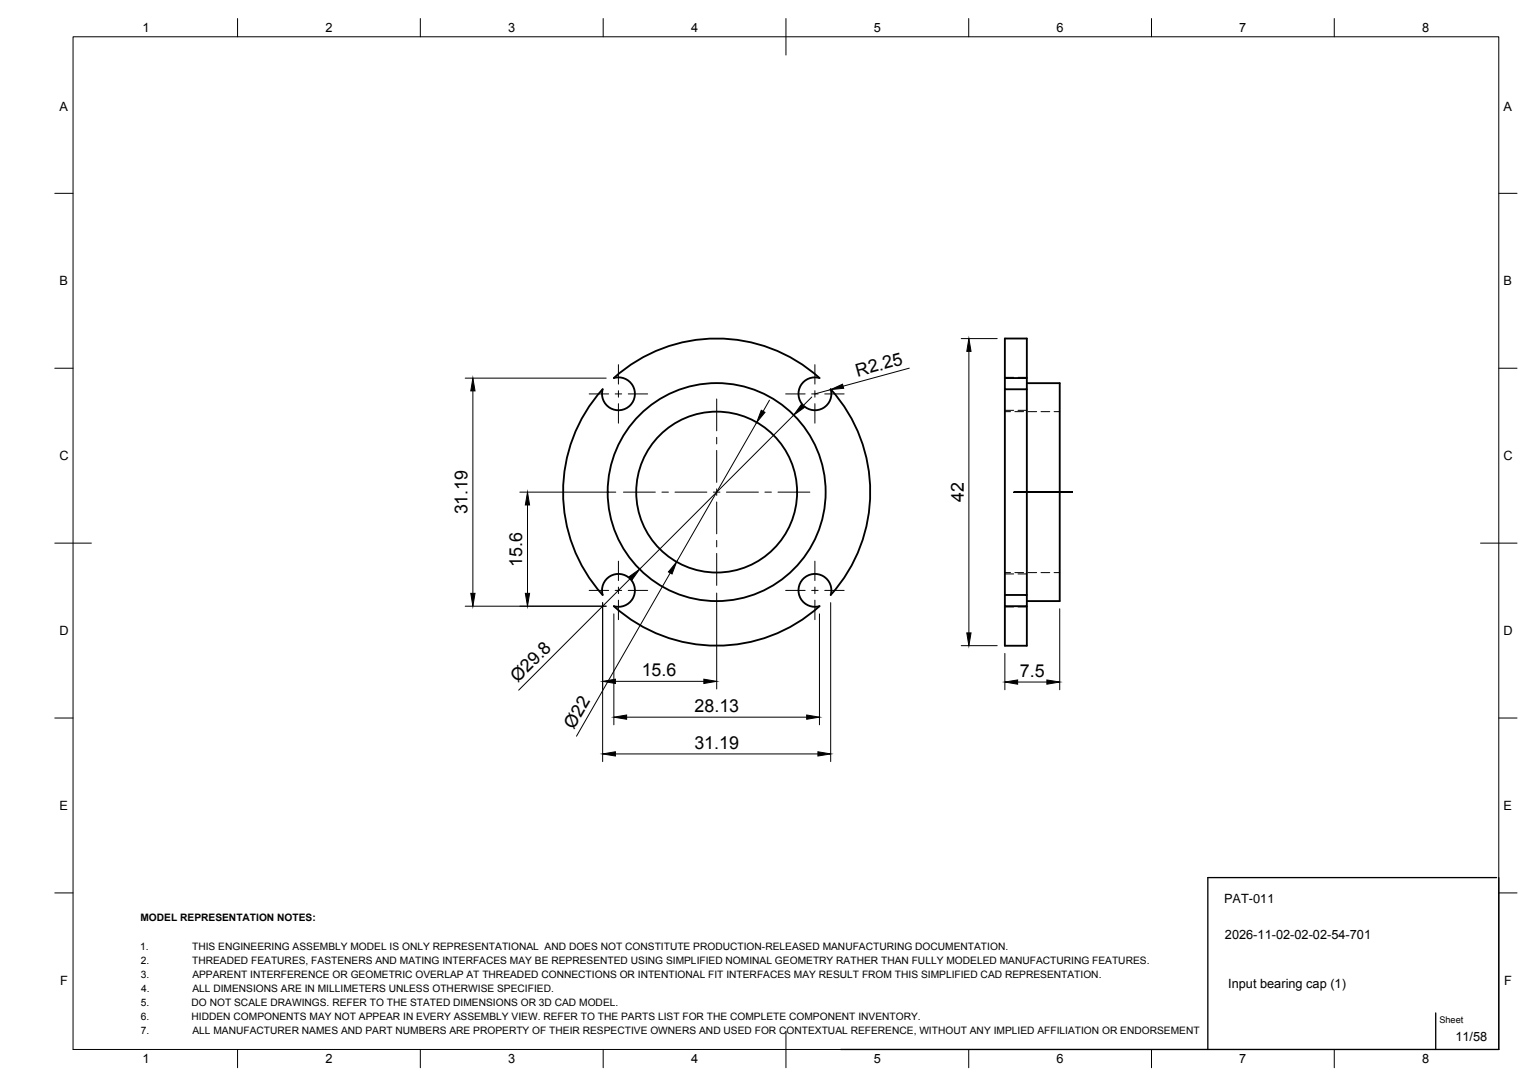
ISO-10303-21;
HEADER;
/* Generated by software containing ST-Developer
 * from STEP Tools, Inc. (www.steptools.com) 
 */

FILE_DESCRIPTION(
/* description */ ('Belt tension measurement rig'),
/* implementation_level */ '2;1');

FILE_NAME(
/* name */ 'Input bearing cap (1).step',
/* time_stamp */ '2026-10-28T03:24:44-07:00',
/* author */ (''),
/* organization */ (''),
/* preprocessor_version */ 'ST-DEVELOPER v20.2',
/* originating_system */ 'Autodesk Translation Framework v15.17.0.0',
/* authorisation */ '');

FILE_SCHEMA (('AUTOMOTIVE_DESIGN { 1 0 10303 214 3 1 1 }'));
ENDSEC;

DATA;
#10=MECHANICAL_DESIGN_GEOMETRIC_PRESENTATION_REPRESENTATION('',(#698),#23587);
#588=SHAPE_REPRESENTATION_RELATIONSHIP('SRR','None',#23833,#643);
#643=ADVANCED_BREP_SHAPE_REPRESENTATION('',(#768),#23531);
#698=STYLED_ITEM('',(#24211),#768);
#768=MANIFOLD_SOLID_BREP('Body1',#12203);
#866=FACE_BOUND('',#2180,.T.);
#867=FACE_BOUND('',#2187,.T.);
#868=FACE_BOUND('',#2190,.T.);
#1084=PLANE('',#13049);
#1085=PLANE('',#13065);
#1086=PLANE('',#13069);
#1434=FACE_OUTER_BOUND('',#2175,.T.);
#1435=FACE_OUTER_BOUND('',#2176,.T.);
#1436=FACE_OUTER_BOUND('',#2177,.T.);
#1437=FACE_OUTER_BOUND('',#2178,.T.);
#1438=FACE_OUTER_BOUND('',#2179,.T.);
#1439=FACE_OUTER_BOUND('',#2181,.T.);
#1440=FACE_OUTER_BOUND('',#2182,.T.);
#1441=FACE_OUTER_BOUND('',#2183,.T.);
#1442=FACE_OUTER_BOUND('',#2184,.T.);
#1443=FACE_OUTER_BOUND('',#2185,.T.);
#1444=FACE_OUTER_BOUND('',#2186,.T.);
#1445=FACE_OUTER_BOUND('',#2188,.T.);
#1446=FACE_OUTER_BOUND('',#2189,.T.);
#2175=EDGE_LOOP('',(#8268,#8269,#8270,#8271));
#2176=EDGE_LOOP('',(#8272,#8273,#8274,#8275));
#2177=EDGE_LOOP('',(#8276,#8277,#8278,#8279));
#2178=EDGE_LOOP('',(#8280,#8281,#8282,#8283));
#2179=EDGE_LOOP('',(#8284,#8285,#8286,#8287,#8288,#8289,#8290,#8291));
#2180=EDGE_LOOP('',(#8292));
#2181=EDGE_LOOP('',(#8293,#8294,#8295,#8296));
#2182=EDGE_LOOP('',(#8297,#8298,#8299,#8300));
#2183=EDGE_LOOP('',(#8301,#8302,#8303,#8304));
#2184=EDGE_LOOP('',(#8305,#8306,#8307,#8308));
#2185=EDGE_LOOP('',(#8309,#8310,#8311,#8312));
#2186=EDGE_LOOP('',(#8313));
#2187=EDGE_LOOP('',(#8314));
#2188=EDGE_LOOP('',(#8315,#8316,#8317,#8318));
#2189=EDGE_LOOP('',(#8319,#8320,#8321,#8322,#8323,#8324,#8325,#8326));
#2190=EDGE_LOOP('',(#8327));
#3063=LINE('',#18919,#3814);
#3064=LINE('',#18923,#3815);
#3065=LINE('',#18928,#3816);
#3066=LINE('',#18932,#3817);
#3067=LINE('',#18937,#3818);
#3068=LINE('',#18941,#3819);
#3069=LINE('',#18946,#3820);
#3070=LINE('',#18950,#3821);
#3071=LINE('',#18969,#3822);
#3072=LINE('',#18977,#3823);
#3814=VECTOR('',#14936,1.);
#3815=VECTOR('',#14939,1.);
#3816=VECTOR('',#14944,1.);
#3817=VECTOR('',#14947,1.);
#3818=VECTOR('',#14952,1.);
#3819=VECTOR('',#14955,1.);
#3820=VECTOR('',#14960,1.);
#3821=VECTOR('',#14963,1.);
#3822=VECTOR('',#14996,1.49);
#3823=VECTOR('',#15007,1.1);
#4540=CIRCLE('',#13038,0.225);
#4541=CIRCLE('',#13039,0.225);
#4542=CIRCLE('',#13041,0.225);
#4543=CIRCLE('',#13042,0.225);
#4544=CIRCLE('',#13044,0.225);
#4545=CIRCLE('',#13045,0.225);
#4546=CIRCLE('',#13047,0.225);
#4547=CIRCLE('',#13048,0.225);
#4548=CIRCLE('',#13050,2.1);
#4549=CIRCLE('',#13051,2.1);
#4550=CIRCLE('',#13052,2.1);
#4551=CIRCLE('',#13053,2.1);
#4552=CIRCLE('',#13054,1.49);
#4553=CIRCLE('',#13056,2.1);
#4554=CIRCLE('',#13058,2.1);
#4555=CIRCLE('',#13060,2.1);
#4556=CIRCLE('',#13062,2.1);
#4557=CIRCLE('',#13064,1.49);
#4558=CIRCLE('',#13066,1.1);
#4559=CIRCLE('',#13068,1.1);
#5348=VERTEX_POINT('',#18917);
#5349=VERTEX_POINT('',#18918);
#5350=VERTEX_POINT('',#18920);
#5351=VERTEX_POINT('',#18922);
#5352=VERTEX_POINT('',#18926);
#5353=VERTEX_POINT('',#18927);
#5354=VERTEX_POINT('',#18929);
#5355=VERTEX_POINT('',#18931);
#5356=VERTEX_POINT('',#18935);
#5357=VERTEX_POINT('',#18936);
#5358=VERTEX_POINT('',#18938);
#5359=VERTEX_POINT('',#18940);
#5360=VERTEX_POINT('',#18944);
#5361=VERTEX_POINT('',#18945);
#5362=VERTEX_POINT('',#18947);
#5363=VERTEX_POINT('',#18949);
#5364=VERTEX_POINT('',#18957);
#5365=VERTEX_POINT('',#18968);
#5366=VERTEX_POINT('',#18972);
#5367=VERTEX_POINT('',#18975);
#6493=EDGE_CURVE('',#5348,#5349,#3063,.T.);
#6494=EDGE_CURVE('',#5350,#5348,#4540,.T.);
#6495=EDGE_CURVE('',#5351,#5350,#3064,.T.);
#6496=EDGE_CURVE('',#5349,#5351,#4541,.T.);
#6497=EDGE_CURVE('',#5352,#5353,#3065,.T.);
#6498=EDGE_CURVE('',#5354,#5352,#4542,.T.);
#6499=EDGE_CURVE('',#5355,#5354,#3066,.T.);
#6500=EDGE_CURVE('',#5353,#5355,#4543,.T.);
#6501=EDGE_CURVE('',#5356,#5357,#3067,.T.);
#6502=EDGE_CURVE('',#5358,#5356,#4544,.T.);
#6503=EDGE_CURVE('',#5359,#5358,#3068,.T.);
#6504=EDGE_CURVE('',#5357,#5359,#4545,.T.);
#6505=EDGE_CURVE('',#5360,#5361,#3069,.T.);
#6506=EDGE_CURVE('',#5362,#5360,#4546,.T.);
#6507=EDGE_CURVE('',#5363,#5362,#3070,.T.);
#6508=EDGE_CURVE('',#5361,#5363,#4547,.T.);
#6509=EDGE_CURVE('',#5362,#5348,#4548,.T.);
#6510=EDGE_CURVE('',#5358,#5360,#4549,.T.);
#6511=EDGE_CURVE('',#5354,#5356,#4550,.T.);
#6512=EDGE_CURVE('',#5350,#5352,#4551,.T.);
#6513=EDGE_CURVE('',#5364,#5364,#4552,.T.);
#6514=EDGE_CURVE('',#5359,#5361,#4553,.T.);
#6515=EDGE_CURVE('',#5355,#5357,#4554,.T.);
#6516=EDGE_CURVE('',#5363,#5349,#4555,.T.);
#6517=EDGE_CURVE('',#5351,#5353,#4556,.T.);
#6518=EDGE_CURVE('',#5364,#5365,#3071,.T.);
#6519=EDGE_CURVE('',#5365,#5365,#4557,.T.);
#6520=EDGE_CURVE('',#5366,#5366,#4558,.T.);
#6521=EDGE_CURVE('',#5367,#5367,#4559,.T.);
#6522=EDGE_CURVE('',#5367,#5366,#3072,.T.);
#8268=ORIENTED_EDGE('',*,*,#6493,.F.);
#8269=ORIENTED_EDGE('',*,*,#6494,.F.);
#8270=ORIENTED_EDGE('',*,*,#6495,.F.);
#8271=ORIENTED_EDGE('',*,*,#6496,.F.);
#8272=ORIENTED_EDGE('',*,*,#6497,.F.);
#8273=ORIENTED_EDGE('',*,*,#6498,.F.);
#8274=ORIENTED_EDGE('',*,*,#6499,.F.);
#8275=ORIENTED_EDGE('',*,*,#6500,.F.);
#8276=ORIENTED_EDGE('',*,*,#6501,.F.);
#8277=ORIENTED_EDGE('',*,*,#6502,.F.);
#8278=ORIENTED_EDGE('',*,*,#6503,.F.);
#8279=ORIENTED_EDGE('',*,*,#6504,.F.);
#8280=ORIENTED_EDGE('',*,*,#6505,.F.);
#8281=ORIENTED_EDGE('',*,*,#6506,.F.);
#8282=ORIENTED_EDGE('',*,*,#6507,.F.);
#8283=ORIENTED_EDGE('',*,*,#6508,.F.);
#8284=ORIENTED_EDGE('',*,*,#6494,.T.);
#8285=ORIENTED_EDGE('',*,*,#6509,.F.);
#8286=ORIENTED_EDGE('',*,*,#6506,.T.);
#8287=ORIENTED_EDGE('',*,*,#6510,.F.);
#8288=ORIENTED_EDGE('',*,*,#6502,.T.);
#8289=ORIENTED_EDGE('',*,*,#6511,.F.);
#8290=ORIENTED_EDGE('',*,*,#6498,.T.);
#8291=ORIENTED_EDGE('',*,*,#6512,.F.);
#8292=ORIENTED_EDGE('',*,*,#6513,.T.);
#8293=ORIENTED_EDGE('',*,*,#6503,.T.);
#8294=ORIENTED_EDGE('',*,*,#6510,.T.);
#8295=ORIENTED_EDGE('',*,*,#6505,.T.);
#8296=ORIENTED_EDGE('',*,*,#6514,.F.);
#8297=ORIENTED_EDGE('',*,*,#6499,.T.);
#8298=ORIENTED_EDGE('',*,*,#6511,.T.);
#8299=ORIENTED_EDGE('',*,*,#6501,.T.);
#8300=ORIENTED_EDGE('',*,*,#6515,.F.);
#8301=ORIENTED_EDGE('',*,*,#6493,.T.);
#8302=ORIENTED_EDGE('',*,*,#6516,.F.);
#8303=ORIENTED_EDGE('',*,*,#6507,.T.);
#8304=ORIENTED_EDGE('',*,*,#6509,.T.);
#8305=ORIENTED_EDGE('',*,*,#6495,.T.);
#8306=ORIENTED_EDGE('',*,*,#6512,.T.);
#8307=ORIENTED_EDGE('',*,*,#6497,.T.);
#8308=ORIENTED_EDGE('',*,*,#6517,.F.);
#8309=ORIENTED_EDGE('',*,*,#6513,.F.);
#8310=ORIENTED_EDGE('',*,*,#6518,.T.);
#8311=ORIENTED_EDGE('',*,*,#6519,.T.);
#8312=ORIENTED_EDGE('',*,*,#6518,.F.);
#8313=ORIENTED_EDGE('',*,*,#6519,.F.);
#8314=ORIENTED_EDGE('',*,*,#6520,.F.);
#8315=ORIENTED_EDGE('',*,*,#6521,.F.);
#8316=ORIENTED_EDGE('',*,*,#6522,.T.);
#8317=ORIENTED_EDGE('',*,*,#6520,.T.);
#8318=ORIENTED_EDGE('',*,*,#6522,.F.);
#8319=ORIENTED_EDGE('',*,*,#6496,.T.);
#8320=ORIENTED_EDGE('',*,*,#6517,.T.);
#8321=ORIENTED_EDGE('',*,*,#6500,.T.);
#8322=ORIENTED_EDGE('',*,*,#6515,.T.);
#8323=ORIENTED_EDGE('',*,*,#6504,.T.);
#8324=ORIENTED_EDGE('',*,*,#6514,.T.);
#8325=ORIENTED_EDGE('',*,*,#6508,.T.);
#8326=ORIENTED_EDGE('',*,*,#6516,.T.);
#8327=ORIENTED_EDGE('',*,*,#6521,.T.);
#11193=CYLINDRICAL_SURFACE('',#13037,0.225);
#11194=CYLINDRICAL_SURFACE('',#13040,0.225);
#11195=CYLINDRICAL_SURFACE('',#13043,0.225);
#11196=CYLINDRICAL_SURFACE('',#13046,0.225);
#11197=CYLINDRICAL_SURFACE('',#13055,2.1);
#11198=CYLINDRICAL_SURFACE('',#13057,2.1);
#11199=CYLINDRICAL_SURFACE('',#13059,2.1);
#11200=CYLINDRICAL_SURFACE('',#13061,2.1);
#11201=CYLINDRICAL_SURFACE('',#13063,1.49);
#11202=CYLINDRICAL_SURFACE('',#13067,1.1);
#11575=ADVANCED_FACE('',(#1434),#11193,.F.);
#11576=ADVANCED_FACE('',(#1435),#11194,.F.);
#11577=ADVANCED_FACE('',(#1436),#11195,.F.);
#11578=ADVANCED_FACE('',(#1437),#11196,.F.);
#11579=ADVANCED_FACE('',(#1438,#866),#1084,.F.);
#11580=ADVANCED_FACE('',(#1439),#11197,.T.);
#11581=ADVANCED_FACE('',(#1440),#11198,.T.);
#11582=ADVANCED_FACE('',(#1441),#11199,.T.);
#11583=ADVANCED_FACE('',(#1442),#11200,.T.);
#11584=ADVANCED_FACE('',(#1443),#11201,.T.);
#11585=ADVANCED_FACE('',(#1444,#867),#1085,.F.);
#11586=ADVANCED_FACE('',(#1445),#11202,.F.);
#11587=ADVANCED_FACE('',(#1446,#868),#1086,.T.);
#12203=CLOSED_SHELL('',(#11575,#11576,#11577,#11578,#11579,#11580,#11581,
#11582,#11583,#11584,#11585,#11586,#11587));
#13036=AXIS2_PLACEMENT_3D('',#18915,#14932,#14933);
#13037=AXIS2_PLACEMENT_3D('',#18916,#14934,#14935);
#13038=AXIS2_PLACEMENT_3D('',#18921,#14937,#14938);
#13039=AXIS2_PLACEMENT_3D('',#18924,#14940,#14941);
#13040=AXIS2_PLACEMENT_3D('',#18925,#14942,#14943);
#13041=AXIS2_PLACEMENT_3D('',#18930,#14945,#14946);
#13042=AXIS2_PLACEMENT_3D('',#18933,#14948,#14949);
#13043=AXIS2_PLACEMENT_3D('',#18934,#14950,#14951);
#13044=AXIS2_PLACEMENT_3D('',#18939,#14953,#14954);
#13045=AXIS2_PLACEMENT_3D('',#18942,#14956,#14957);
#13046=AXIS2_PLACEMENT_3D('',#18943,#14958,#14959);
#13047=AXIS2_PLACEMENT_3D('',#18948,#14961,#14962);
#13048=AXIS2_PLACEMENT_3D('',#18951,#14964,#14965);
#13049=AXIS2_PLACEMENT_3D('',#18952,#14966,#14967);
#13050=AXIS2_PLACEMENT_3D('',#18953,#14968,#14969);
#13051=AXIS2_PLACEMENT_3D('',#18954,#14970,#14971);
#13052=AXIS2_PLACEMENT_3D('',#18955,#14972,#14973);
#13053=AXIS2_PLACEMENT_3D('',#18956,#14974,#14975);
#13054=AXIS2_PLACEMENT_3D('',#18958,#14976,#14977);
#13055=AXIS2_PLACEMENT_3D('',#18959,#14978,#14979);
#13056=AXIS2_PLACEMENT_3D('',#18960,#14980,#14981);
#13057=AXIS2_PLACEMENT_3D('',#18961,#14982,#14983);
#13058=AXIS2_PLACEMENT_3D('',#18962,#14984,#14985);
#13059=AXIS2_PLACEMENT_3D('',#18963,#14986,#14987);
#13060=AXIS2_PLACEMENT_3D('',#18964,#14988,#14989);
#13061=AXIS2_PLACEMENT_3D('',#18965,#14990,#14991);
#13062=AXIS2_PLACEMENT_3D('',#18966,#14992,#14993);
#13063=AXIS2_PLACEMENT_3D('',#18967,#14994,#14995);
#13064=AXIS2_PLACEMENT_3D('',#18970,#14997,#14998);
#13065=AXIS2_PLACEMENT_3D('',#18971,#14999,#15000);
#13066=AXIS2_PLACEMENT_3D('',#18973,#15001,#15002);
#13067=AXIS2_PLACEMENT_3D('',#18974,#15003,#15004);
#13068=AXIS2_PLACEMENT_3D('',#18976,#15005,#15006);
#13069=AXIS2_PLACEMENT_3D('',#18978,#15008,#15009);
#14932=DIRECTION('axis',(0.,0.,1.));
#14933=DIRECTION('refdir',(1.,0.,0.));
#14934=DIRECTION('center_axis',(0.,1.,0.));
#14935=DIRECTION('ref_axis',(0.707106781186546,0.,0.707106781186549));
#14936=DIRECTION('',(0.,1.,0.));
#14937=DIRECTION('center_axis',(0.,1.,0.));
#14938=DIRECTION('ref_axis',(1.,0.,0.));
#14939=DIRECTION('',(0.,-1.,0.));
#14940=DIRECTION('center_axis',(0.,-1.,0.));
#14941=DIRECTION('ref_axis',(1.,0.,0.));
#14942=DIRECTION('center_axis',(0.,1.,0.));
#14943=DIRECTION('ref_axis',(0.707106781186547,0.,-0.707106781186548));
#14944=DIRECTION('',(0.,1.,0.));
#14945=DIRECTION('center_axis',(0.,1.,0.));
#14946=DIRECTION('ref_axis',(1.,0.,0.));
#14947=DIRECTION('',(0.,-1.,0.));
#14948=DIRECTION('center_axis',(0.,-1.,0.));
#14949=DIRECTION('ref_axis',(1.,0.,0.));
#14950=DIRECTION('center_axis',(0.,1.,0.));
#14951=DIRECTION('ref_axis',(-0.707106781186552,0.,-0.707106781186543));
#14952=DIRECTION('',(0.,1.,0.));
#14953=DIRECTION('center_axis',(0.,1.,0.));
#14954=DIRECTION('ref_axis',(1.,0.,0.));
#14955=DIRECTION('',(0.,-1.,0.));
#14956=DIRECTION('center_axis',(0.,-1.,0.));
#14957=DIRECTION('ref_axis',(1.,0.,0.));
#14958=DIRECTION('center_axis',(0.,1.,0.));
#14959=DIRECTION('ref_axis',(-0.707106781186546,0.,0.707106781186549));
#14960=DIRECTION('',(0.,1.,0.));
#14961=DIRECTION('center_axis',(0.,1.,0.));
#14962=DIRECTION('ref_axis',(1.,0.,0.));
#14963=DIRECTION('',(0.,-1.,0.));
#14964=DIRECTION('center_axis',(0.,-1.,0.));
#14965=DIRECTION('ref_axis',(1.,0.,0.));
#14966=DIRECTION('center_axis',(0.,1.,0.));
#14967=DIRECTION('ref_axis',(1.,0.,0.));
#14968=DIRECTION('center_axis',(0.,1.,0.));
#14969=DIRECTION('ref_axis',(1.,0.,0.));
#14970=DIRECTION('center_axis',(0.,1.,0.));
#14971=DIRECTION('ref_axis',(1.,0.,0.));
#14972=DIRECTION('center_axis',(0.,1.,0.));
#14973=DIRECTION('ref_axis',(1.,0.,0.));
#14974=DIRECTION('center_axis',(0.,1.,0.));
#14975=DIRECTION('ref_axis',(1.,0.,0.));
#14976=DIRECTION('center_axis',(0.,1.,0.));
#14977=DIRECTION('ref_axis',(1.,0.,0.));
#14978=DIRECTION('center_axis',(0.,1.,0.));
#14979=DIRECTION('ref_axis',(1.,0.,0.));
#14980=DIRECTION('center_axis',(0.,1.,0.));
#14981=DIRECTION('ref_axis',(1.,0.,0.));
#14982=DIRECTION('center_axis',(0.,1.,0.));
#14983=DIRECTION('ref_axis',(1.,0.,0.));
#14984=DIRECTION('center_axis',(0.,1.,0.));
#14985=DIRECTION('ref_axis',(1.,0.,0.));
#14986=DIRECTION('center_axis',(0.,1.,0.));
#14987=DIRECTION('ref_axis',(1.,0.,0.));
#14988=DIRECTION('center_axis',(0.,1.,0.));
#14989=DIRECTION('ref_axis',(1.,0.,0.));
#14990=DIRECTION('center_axis',(0.,1.,0.));
#14991=DIRECTION('ref_axis',(-1.,0.,-1.22464679914735E-16));
#14992=DIRECTION('center_axis',(0.,1.,0.));
#14993=DIRECTION('ref_axis',(1.,0.,0.));
#14994=DIRECTION('center_axis',(0.,1.,0.));
#14995=DIRECTION('ref_axis',(1.,0.,0.));
#14996=DIRECTION('',(0.,-1.,0.));
#14997=DIRECTION('center_axis',(0.,1.,0.));
#14998=DIRECTION('ref_axis',(1.,0.,0.));
#14999=DIRECTION('center_axis',(0.,1.,0.));
#15000=DIRECTION('ref_axis',(1.,0.,0.));
#15001=DIRECTION('center_axis',(0.,-1.,0.));
#15002=DIRECTION('ref_axis',(1.,0.,0.));
#15003=DIRECTION('center_axis',(0.,1.,0.));
#15004=DIRECTION('ref_axis',(1.,0.,0.));
#15005=DIRECTION('center_axis',(0.,-1.,0.));
#15006=DIRECTION('ref_axis',(1.,0.,0.));
#15007=DIRECTION('',(0.,-1.,0.));
#15008=DIRECTION('center_axis',(0.,1.,0.));
#15009=DIRECTION('ref_axis',(1.,0.,0.));
#18915=CARTESIAN_POINT('',(0.,0.,0.));
#18916=CARTESIAN_POINT('Origin',(-1.34350288425444,1.7,5.65649711574556));
#18917=CARTESIAN_POINT('',(-1.40634555589641,1.8,5.4404512904656));
#18918=CARTESIAN_POINT('',(-1.40634555589641,2.1,5.4404512904656));
#18919=CARTESIAN_POINT('',(-1.40634555589641,1.7,5.4404512904656));
#18920=CARTESIAN_POINT('',(-1.5595487095344,1.8,5.59365444410359));
#18921=CARTESIAN_POINT('Origin',(-1.34350288425444,1.8,5.65649711574556));
#18922=CARTESIAN_POINT('',(-1.5595487095344,2.1,5.59365444410359));
#18923=CARTESIAN_POINT('',(-1.5595487095344,1.7,5.59365444410359));
#18924=CARTESIAN_POINT('Origin',(-1.34350288425444,2.1,5.65649711574556));
#18925=CARTESIAN_POINT('Origin',(-1.34350288425444,1.7,8.34350288425444));
#18926=CARTESIAN_POINT('',(-1.5595487095344,1.8,8.40634555589641));
#18927=CARTESIAN_POINT('',(-1.5595487095344,2.1,8.40634555589641));
#18928=CARTESIAN_POINT('',(-1.5595487095344,1.7,8.40634555589641));
#18929=CARTESIAN_POINT('',(-1.40634555589641,1.8,8.5595487095344));
#18930=CARTESIAN_POINT('Origin',(-1.34350288425444,1.8,8.34350288425444));
#18931=CARTESIAN_POINT('',(-1.40634555589641,2.1,8.5595487095344));
#18932=CARTESIAN_POINT('',(-1.40634555589641,1.7,8.5595487095344));
#18933=CARTESIAN_POINT('Origin',(-1.34350288425444,2.1,8.34350288425444));
#18934=CARTESIAN_POINT('Origin',(1.34350288425444,1.7,8.34350288425444));
#18935=CARTESIAN_POINT('',(1.40634555589641,1.8,8.5595487095344));
#18936=CARTESIAN_POINT('',(1.40634555589641,2.1,8.5595487095344));
#18937=CARTESIAN_POINT('',(1.40634555589641,1.7,8.5595487095344));
#18938=CARTESIAN_POINT('',(1.5595487095344,1.8,8.40634555589641));
#18939=CARTESIAN_POINT('Origin',(1.34350288425444,1.8,8.34350288425444));
#18940=CARTESIAN_POINT('',(1.5595487095344,2.1,8.40634555589641));
#18941=CARTESIAN_POINT('',(1.5595487095344,1.7,8.40634555589641));
#18942=CARTESIAN_POINT('Origin',(1.34350288425444,2.1,8.34350288425444));
#18943=CARTESIAN_POINT('Origin',(1.34350288425444,1.7,5.65649711574556));
#18944=CARTESIAN_POINT('',(1.5595487095344,1.8,5.59365444410359));
#18945=CARTESIAN_POINT('',(1.5595487095344,2.1,5.59365444410359));
#18946=CARTESIAN_POINT('',(1.5595487095344,1.7,5.59365444410359));
#18947=CARTESIAN_POINT('',(1.40634555589641,1.8,5.4404512904656));
#18948=CARTESIAN_POINT('Origin',(1.34350288425444,1.8,5.65649711574556));
#18949=CARTESIAN_POINT('',(1.40634555589641,2.1,5.4404512904656));
#18950=CARTESIAN_POINT('',(1.40634555589641,1.7,5.4404512904656));
#18951=CARTESIAN_POINT('Origin',(1.34350288425444,2.1,5.65649711574556));
#18952=CARTESIAN_POINT('Origin',(0.,1.8,7.));
#18953=CARTESIAN_POINT('Origin',(0.,1.8,7.));
#18954=CARTESIAN_POINT('Origin',(0.,1.8,7.));
#18955=CARTESIAN_POINT('Origin',(0.,1.8,7.));
#18956=CARTESIAN_POINT('Origin',(0.,1.8,7.));
#18957=CARTESIAN_POINT('',(-1.49,1.8,7.));
#18958=CARTESIAN_POINT('Origin',(0.,1.8,7.));
#18959=CARTESIAN_POINT('Origin',(0.,1.8,7.));
#18960=CARTESIAN_POINT('Origin',(0.,2.1,7.));
#18961=CARTESIAN_POINT('Origin',(0.,1.8,7.));
#18962=CARTESIAN_POINT('Origin',(0.,2.1,7.));
#18963=CARTESIAN_POINT('Origin',(0.,1.8,7.));
#18964=CARTESIAN_POINT('Origin',(0.,2.1,7.));
#18965=CARTESIAN_POINT('Origin',(0.,1.8,7.));
#18966=CARTESIAN_POINT('Origin',(0.,2.1,7.));
#18967=CARTESIAN_POINT('Origin',(0.,1.35,7.));
#18968=CARTESIAN_POINT('',(-1.49,1.35,7.));
#18969=CARTESIAN_POINT('',(-1.49,1.35,7.));
#18970=CARTESIAN_POINT('Origin',(0.,1.35,7.));
#18971=CARTESIAN_POINT('Origin',(0.,1.35,7.));
#18972=CARTESIAN_POINT('',(-1.1,1.35,7.));
#18973=CARTESIAN_POINT('Origin',(0.,1.35,7.));
#18974=CARTESIAN_POINT('Origin',(0.,1.8,7.));
#18975=CARTESIAN_POINT('',(-1.1,2.1,7.));
#18976=CARTESIAN_POINT('Origin',(0.,2.1,7.));
#18977=CARTESIAN_POINT('',(-1.1,1.8,7.));
#18978=CARTESIAN_POINT('Origin',(0.,2.1,7.));
#23466=UNCERTAINTY_MEASURE_WITH_UNIT(LENGTH_MEASURE(0.001),#23588,
'DISTANCE_ACCURACY_VALUE',
'Maximum model space distance between geometric entities at asserted c
onnectivities');
#23522=UNCERTAINTY_MEASURE_WITH_UNIT(LENGTH_MEASURE(0.001),#23588,
'DISTANCE_ACCURACY_VALUE',
'Maximum model space distance between geometric entities at asserted c
onnectivities');
#23531=(
GEOMETRIC_REPRESENTATION_CONTEXT(3)
GLOBAL_UNCERTAINTY_ASSIGNED_CONTEXT((#23466))
GLOBAL_UNIT_ASSIGNED_CONTEXT((#23588,#23590,#23591))
REPRESENTATION_CONTEXT('','3D')
);
#23587=(
GEOMETRIC_REPRESENTATION_CONTEXT(3)
GLOBAL_UNCERTAINTY_ASSIGNED_CONTEXT((#23522))
GLOBAL_UNIT_ASSIGNED_CONTEXT((#23588,#23590,#23591))
REPRESENTATION_CONTEXT('','3D')
);
#23588=(
LENGTH_UNIT()
NAMED_UNIT(*)
SI_UNIT(.CENTI.,.METRE.)
);
#23590=(
NAMED_UNIT(*)
PLANE_ANGLE_UNIT()
SI_UNIT($,.RADIAN.)
);
#23591=(
NAMED_UNIT(*)
SI_UNIT($,.STERADIAN.)
SOLID_ANGLE_UNIT()
);
#23600=SHAPE_DEFINITION_REPRESENTATION(#23664,#23833);
#23664=PRODUCT_DEFINITION_SHAPE('',$,#23898);
#23833=SHAPE_REPRESENTATION('',(#13036),#23531);
#23889=PRODUCT_DEFINITION_CONTEXT('part definition',#24083,'design');
#23898=PRODUCT_DEFINITION('Input bearing cap (1)','Input bearing cap (1)',
#23962,#23889);
#23962=PRODUCT_DEFINITION_FORMATION('',$,#24093);
#24083=APPLICATION_CONTEXT(
'Core Data for Automotive Mechanical Design Process');
#24084=PRODUCT_CONTEXT('part definition',#24083,'mechanical');
#24093=PRODUCT('Input bearing cap (1)','Input bearing cap (1)',
'Input bearing cap (1)',(#24084));
#24205=COLOUR_RGB('Grey',0.48,0.52,0.57);
#24206=FILL_AREA_STYLE_COLOUR('',#24205);
#24207=FILL_AREA_STYLE('',(#24206));
#24208=SURFACE_STYLE_FILL_AREA(#24207);
#24209=SURFACE_SIDE_STYLE('',(#24208));
#24210=SURFACE_STYLE_USAGE(.BOTH.,#24209);
#24211=PRESENTATION_STYLE_ASSIGNMENT((#24210));
ENDSEC;
END-ISO-10303-21;
